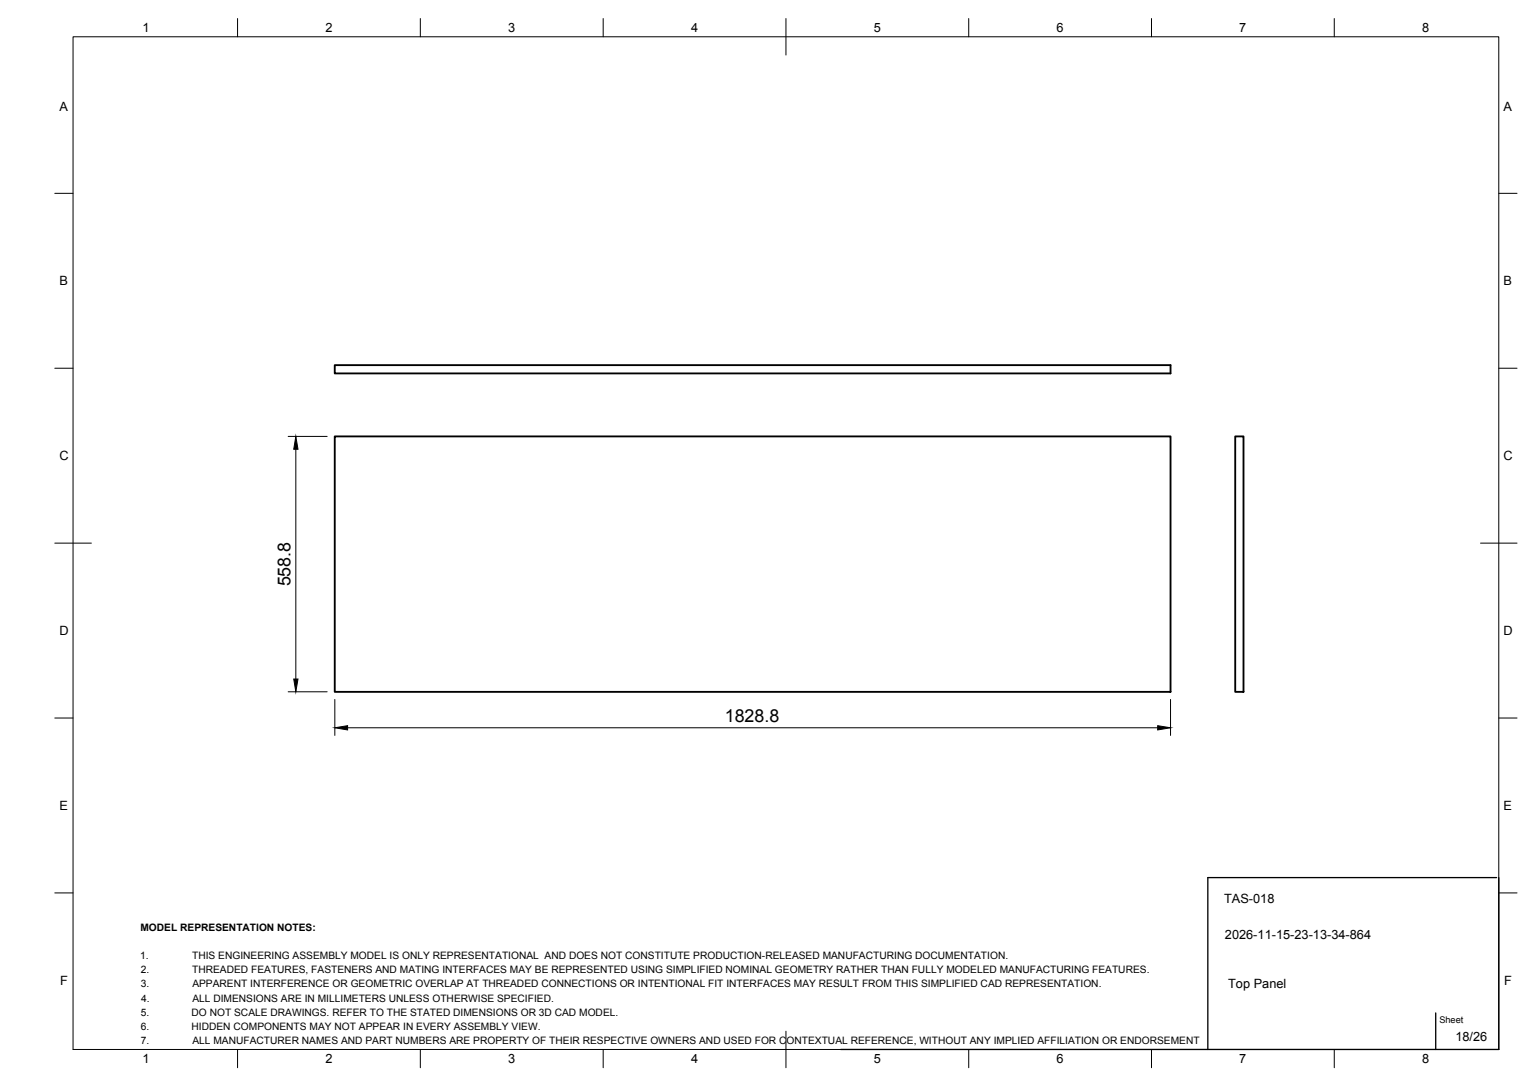
ISO-10303-21;
HEADER;
/* Generated by software containing ST-Developer
 * from STEP Tools, Inc. (www.steptools.com) 
 */

FILE_DESCRIPTION(
/* description */ (''),
/* implementation_level */ '2;1');

FILE_NAME(
/* name */ 'Top Panel.step',
/* time_stamp */ '2026-11-15T15:17:57-08:00',
/* author */ (''),
/* organization */ (''),
/* preprocessor_version */ 'ST-DEVELOPER v20.2',
/* originating_system */ 'Autodesk Translation Framework v15.17.0.0',
/* authorisation */ '');

FILE_SCHEMA (('AUTOMOTIVE_DESIGN { 1 0 10303 214 3 1 1 }'));
ENDSEC;

DATA;
#10=MECHANICAL_DESIGN_GEOMETRIC_PRESENTATION_REPRESENTATION('',(#193),#3723);
#145=SHAPE_REPRESENTATION_RELATIONSHIP('SRR','None',#3826,#169);
#169=ADVANCED_BREP_SHAPE_REPRESENTATION('',(#217),#3715);
#193=STYLED_ITEM('',(#3948),#217);
#217=MANIFOLD_SOLID_BREP('Body1',#2041);
#315=FACE_OUTER_BOUND('',#441,.T.);
#316=FACE_OUTER_BOUND('',#442,.T.);
#317=FACE_OUTER_BOUND('',#443,.T.);
#318=FACE_OUTER_BOUND('',#444,.T.);
#319=FACE_OUTER_BOUND('',#445,.T.);
#320=FACE_OUTER_BOUND('',#446,.T.);
#441=EDGE_LOOP('',(#1659,#1660,#1661,#1662));
#442=EDGE_LOOP('',(#1663,#1664,#1665,#1666));
#443=EDGE_LOOP('',(#1667,#1668,#1669,#1670));
#444=EDGE_LOOP('',(#1671,#1672,#1673,#1674));
#445=EDGE_LOOP('',(#1675,#1676,#1677,#1678));
#446=EDGE_LOOP('',(#1679,#1680,#1681,#1682));
#647=LINE('',#3506,#869);
#648=LINE('',#3508,#870);
#649=LINE('',#3510,#871);
#650=LINE('',#3511,#872);
#651=LINE('',#3514,#873);
#652=LINE('',#3516,#874);
#653=LINE('',#3517,#875);
#654=LINE('',#3520,#876);
#655=LINE('',#3522,#877);
#656=LINE('',#3523,#878);
#657=LINE('',#3525,#879);
#658=LINE('',#3526,#880);
#869=VECTOR('',#2903,22.);
#870=VECTOR('',#2904,0.708661417322828);
#871=VECTOR('',#2905,22.);
#872=VECTOR('',#2906,0.708661417322828);
#873=VECTOR('',#2909,72.);
#874=VECTOR('',#2910,0.708661417322828);
#875=VECTOR('',#2911,72.);
#876=VECTOR('',#2914,22.);
#877=VECTOR('',#2915,0.708661417322828);
#878=VECTOR('',#2916,22.);
#879=VECTOR('',#2919,72.);
#880=VECTOR('',#2920,72.);
#1037=VERTEX_POINT('',#3504);
#1038=VERTEX_POINT('',#3505);
#1039=VERTEX_POINT('',#3507);
#1040=VERTEX_POINT('',#3509);
#1041=VERTEX_POINT('',#3513);
#1042=VERTEX_POINT('',#3515);
#1043=VERTEX_POINT('',#3519);
#1044=VERTEX_POINT('',#3521);
#1251=EDGE_CURVE('',#1037,#1038,#647,.T.);
#1252=EDGE_CURVE('',#1039,#1038,#648,.T.);
#1253=EDGE_CURVE('',#1040,#1039,#649,.T.);
#1254=EDGE_CURVE('',#1040,#1037,#650,.T.);
#1255=EDGE_CURVE('',#1038,#1041,#651,.T.);
#1256=EDGE_CURVE('',#1042,#1041,#652,.T.);
#1257=EDGE_CURVE('',#1039,#1042,#653,.T.);
#1258=EDGE_CURVE('',#1041,#1043,#654,.T.);
#1259=EDGE_CURVE('',#1044,#1043,#655,.T.);
#1260=EDGE_CURVE('',#1042,#1044,#656,.T.);
#1261=EDGE_CURVE('',#1043,#1037,#657,.T.);
#1262=EDGE_CURVE('',#1044,#1040,#658,.T.);
#1659=ORIENTED_EDGE('',*,*,#1251,.T.);
#1660=ORIENTED_EDGE('',*,*,#1252,.F.);
#1661=ORIENTED_EDGE('',*,*,#1253,.F.);
#1662=ORIENTED_EDGE('',*,*,#1254,.T.);
#1663=ORIENTED_EDGE('',*,*,#1255,.T.);
#1664=ORIENTED_EDGE('',*,*,#1256,.F.);
#1665=ORIENTED_EDGE('',*,*,#1257,.F.);
#1666=ORIENTED_EDGE('',*,*,#1252,.T.);
#1667=ORIENTED_EDGE('',*,*,#1258,.T.);
#1668=ORIENTED_EDGE('',*,*,#1259,.F.);
#1669=ORIENTED_EDGE('',*,*,#1260,.F.);
#1670=ORIENTED_EDGE('',*,*,#1256,.T.);
#1671=ORIENTED_EDGE('',*,*,#1261,.T.);
#1672=ORIENTED_EDGE('',*,*,#1254,.F.);
#1673=ORIENTED_EDGE('',*,*,#1262,.F.);
#1674=ORIENTED_EDGE('',*,*,#1259,.T.);
#1675=ORIENTED_EDGE('',*,*,#1253,.T.);
#1676=ORIENTED_EDGE('',*,*,#1257,.T.);
#1677=ORIENTED_EDGE('',*,*,#1260,.T.);
#1678=ORIENTED_EDGE('',*,*,#1262,.T.);
#1679=ORIENTED_EDGE('',*,*,#1251,.F.);
#1680=ORIENTED_EDGE('',*,*,#1261,.F.);
#1681=ORIENTED_EDGE('',*,*,#1258,.F.);
#1682=ORIENTED_EDGE('',*,*,#1255,.F.);
#1867=PLANE('',#2428);
#1868=PLANE('',#2429);
#1869=PLANE('',#2430);
#1870=PLANE('',#2431);
#1871=PLANE('',#2432);
#1872=PLANE('',#2433);
#1989=ADVANCED_FACE('',(#315),#1867,.F.);
#1990=ADVANCED_FACE('',(#316),#1868,.F.);
#1991=ADVANCED_FACE('',(#317),#1869,.F.);
#1992=ADVANCED_FACE('',(#318),#1870,.F.);
#1993=ADVANCED_FACE('',(#319),#1871,.T.);
#1994=ADVANCED_FACE('',(#320),#1872,.F.);
#2041=CLOSED_SHELL('',(#1989,#1990,#1991,#1992,#1993,#1994));
#2427=AXIS2_PLACEMENT_3D('',#3502,#2899,#2900);
#2428=AXIS2_PLACEMENT_3D('',#3503,#2901,#2902);
#2429=AXIS2_PLACEMENT_3D('',#3512,#2907,#2908);
#2430=AXIS2_PLACEMENT_3D('',#3518,#2912,#2913);
#2431=AXIS2_PLACEMENT_3D('',#3524,#2917,#2918);
#2432=AXIS2_PLACEMENT_3D('',#3527,#2921,#2922);
#2433=AXIS2_PLACEMENT_3D('',#3528,#2923,#2924);
#2899=DIRECTION('axis',(0.,0.,1.));
#2900=DIRECTION('refdir',(1.,0.,0.));
#2901=DIRECTION('center_axis',(1.,-1.85037170770859E-14,-1.98679854084674E-16));
#2902=DIRECTION('ref_axis',(-1.98679854084674E-16,0.,-1.));
#2903=DIRECTION('',(0.,0.,1.));
#2904=DIRECTION('',(-2.36847578586702E-14,-1.,0.));
#2905=DIRECTION('',(2.54310213228382E-16,0.,1.));
#2906=DIRECTION('',(-1.57898385724468E-14,-1.,-2.04540917754051E-46));
#2907=DIRECTION('center_axis',(3.77483350043889E-60,2.04540917754051E-46,
-1.));
#2908=DIRECTION('ref_axis',(-1.,0.,-3.77483350043889E-60));
#2909=DIRECTION('',(1.,-1.84940038397751E-14,0.));
#2910=DIRECTION('',(-1.57898385724468E-14,-1.,0.));
#2911=DIRECTION('',(1.,-1.84940038397751E-14,0.));
#2912=DIRECTION('center_axis',(-1.,1.85037170770859E-14,0.));
#2913=DIRECTION('ref_axis',(0.,0.,1.));
#2914=DIRECTION('',(0.,0.,-1.));
#2915=DIRECTION('',(-1.57898385724468E-14,-1.,-2.04540917754051E-46));
#2916=DIRECTION('',(0.,0.,-1.));
#2917=DIRECTION('center_axis',(9.93377236957248E-63,-2.04540917754051E-46,
1.));
#2918=DIRECTION('ref_axis',(1.,0.,-9.93377236957248E-63));
#2919=DIRECTION('',(-1.,1.84940038397751E-14,3.78476727280846E-60));
#2920=DIRECTION('',(-1.,1.84940038397751E-14,3.78432352684346E-60));
#2921=DIRECTION('center_axis',(1.84551508905319E-14,1.,-3.66666668604152E-30));
#2922=DIRECTION('ref_axis',(0.,3.66666668604152E-30,1.));
#2923=DIRECTION('center_axis',(1.84551508905319E-14,1.,-3.66666668604152E-30));
#2924=DIRECTION('ref_axis',(0.,3.66666668604152E-30,1.));
#3502=CARTESIAN_POINT('',(0.,0.,0.));
#3503=CARTESIAN_POINT('Origin',(-36.,80.0000000000007,1.44950256676235E-46));
#3504=CARTESIAN_POINT('',(-36.,79.2913385826778,1.36251621821105E-58));
#3505=CARTESIAN_POINT('',(-36.,79.2913385826778,22.));
#3506=CARTESIAN_POINT('',(-36.,79.2913385826778,1.36251621821105E-58));
#3507=CARTESIAN_POINT('',(-36.,80.0000000000007,22.));
#3508=CARTESIAN_POINT('',(-36.,80.0000000000007,22.));
#3509=CARTESIAN_POINT('',(-36.,80.0000000000007,1.44950256676235E-46));
#3510=CARTESIAN_POINT('',(-36.,80.0000000000007,1.44950256676235E-46));
#3511=CARTESIAN_POINT('',(-36.,80.0000000000007,1.44950256676235E-46));
#3512=CARTESIAN_POINT('Origin',(-36.,80.0000000000007,22.));
#3513=CARTESIAN_POINT('',(36.,79.2913385826765,22.));
#3514=CARTESIAN_POINT('',(-36.,79.2913385826778,22.));
#3515=CARTESIAN_POINT('',(36.,79.9999999999993,22.));
#3516=CARTESIAN_POINT('',(36.,79.9999999999993,22.));
#3517=CARTESIAN_POINT('',(-36.,80.0000000000007,22.));
#3518=CARTESIAN_POINT('Origin',(36.,79.9999999999993,1.44950256675963E-46));
#3519=CARTESIAN_POINT('',(36.,79.2913385826765,-1.36251621821105E-58));
#3520=CARTESIAN_POINT('',(36.,79.2913385826765,22.));
#3521=CARTESIAN_POINT('',(36.,79.9999999999993,1.44950256675963E-46));
#3522=CARTESIAN_POINT('',(36.,79.9999999999993,1.44950256675963E-46));
#3523=CARTESIAN_POINT('',(36.,79.9999999999993,22.));
#3524=CARTESIAN_POINT('Origin',(-36.,80.0000000000007,1.44950256676235E-46));
#3525=CARTESIAN_POINT('',(36.,79.2913385826765,-1.36251621821105E-58));
#3526=CARTESIAN_POINT('',(36.,79.9999999999993,1.44950256675963E-46));
#3527=CARTESIAN_POINT('Origin',(1.47644648822515E-12,80.,-2.90734909672741E-28));
#3528=CARTESIAN_POINT('Origin',(1.46333361785556E-12,79.2913385826772,-2.90734909672741E-28));
#3688=UNCERTAINTY_MEASURE_WITH_UNIT(LENGTH_MEASURE(0.000393700787401575),
#3725,'DISTANCE_ACCURACY_VALUE',
'Maximum model space distance between geometric entities at asserted c
onnectivities');
#3696=UNCERTAINTY_MEASURE_WITH_UNIT(LENGTH_MEASURE(0.000393700787401575),
#3725,'DISTANCE_ACCURACY_VALUE',
'Maximum model space distance between geometric entities at asserted c
onnectivities');
#3715=(
GEOMETRIC_REPRESENTATION_CONTEXT(3)
GLOBAL_UNCERTAINTY_ASSIGNED_CONTEXT((#3688))
GLOBAL_UNIT_ASSIGNED_CONTEXT((#3725,#3729,#3730))
REPRESENTATION_CONTEXT('','3D')
);
#3723=(
GEOMETRIC_REPRESENTATION_CONTEXT(3)
GLOBAL_UNCERTAINTY_ASSIGNED_CONTEXT((#3696))
GLOBAL_UNIT_ASSIGNED_CONTEXT((#3725,#3729,#3730))
REPRESENTATION_CONTEXT('','3D')
);
#3724=DIMENSIONAL_EXPONENTS(1.,0.,0.,0.,0.,0.,0.);
#3725=(
CONVERSION_BASED_UNIT('inch',#3728)
LENGTH_UNIT()
NAMED_UNIT(#3724)
);
#3726=(
LENGTH_UNIT()
NAMED_UNIT(*)
SI_UNIT(.MILLI.,.METRE.)
);
#3728=LENGTH_MEASURE_WITH_UNIT(LENGTH_MEASURE(25.4),#3726);
#3729=(
NAMED_UNIT(*)
PLANE_ANGLE_UNIT()
SI_UNIT($,.RADIAN.)
);
#3730=(
NAMED_UNIT(*)
SI_UNIT($,.STERADIAN.)
SOLID_ANGLE_UNIT()
);
#3749=SHAPE_DEFINITION_REPRESENTATION(#3776,#3826);
#3776=PRODUCT_DEFINITION_SHAPE('',$,#3853);
#3826=SHAPE_REPRESENTATION('',(#2427),#3715);
#3834=PRODUCT_DEFINITION_CONTEXT('part definition',#3914,'design');
#3853=PRODUCT_DEFINITION('2026-11-15-23-13-34-864','Top Panel',#3879,#3834);
#3879=PRODUCT_DEFINITION_FORMATION('',$,#3934);
#3914=APPLICATION_CONTEXT(
'Core Data for Automotive Mechanical Design Process');
#3915=PRODUCT_CONTEXT('part definition',#3914,'mechanical');
#3934=PRODUCT('2026-11-15-23-13-34-864','Top Panel',$,(#3915));
#3948=PRESENTATION_STYLE_ASSIGNMENT((#3956));
#3956=SURFACE_STYLE_USAGE(.BOTH.,#3964);
#3964=SURFACE_SIDE_STYLE('',(#3972));
#3972=SURFACE_STYLE_FILL_AREA(#3980);
#3980=FILL_AREA_STYLE('Blue',(#3988));
#3988=FILL_AREA_STYLE_COLOUR('Blue',#3996);
#3996=COLOUR_RGB('Blue',0.,0.4,0.8);
ENDSEC;
END-ISO-10303-21;
